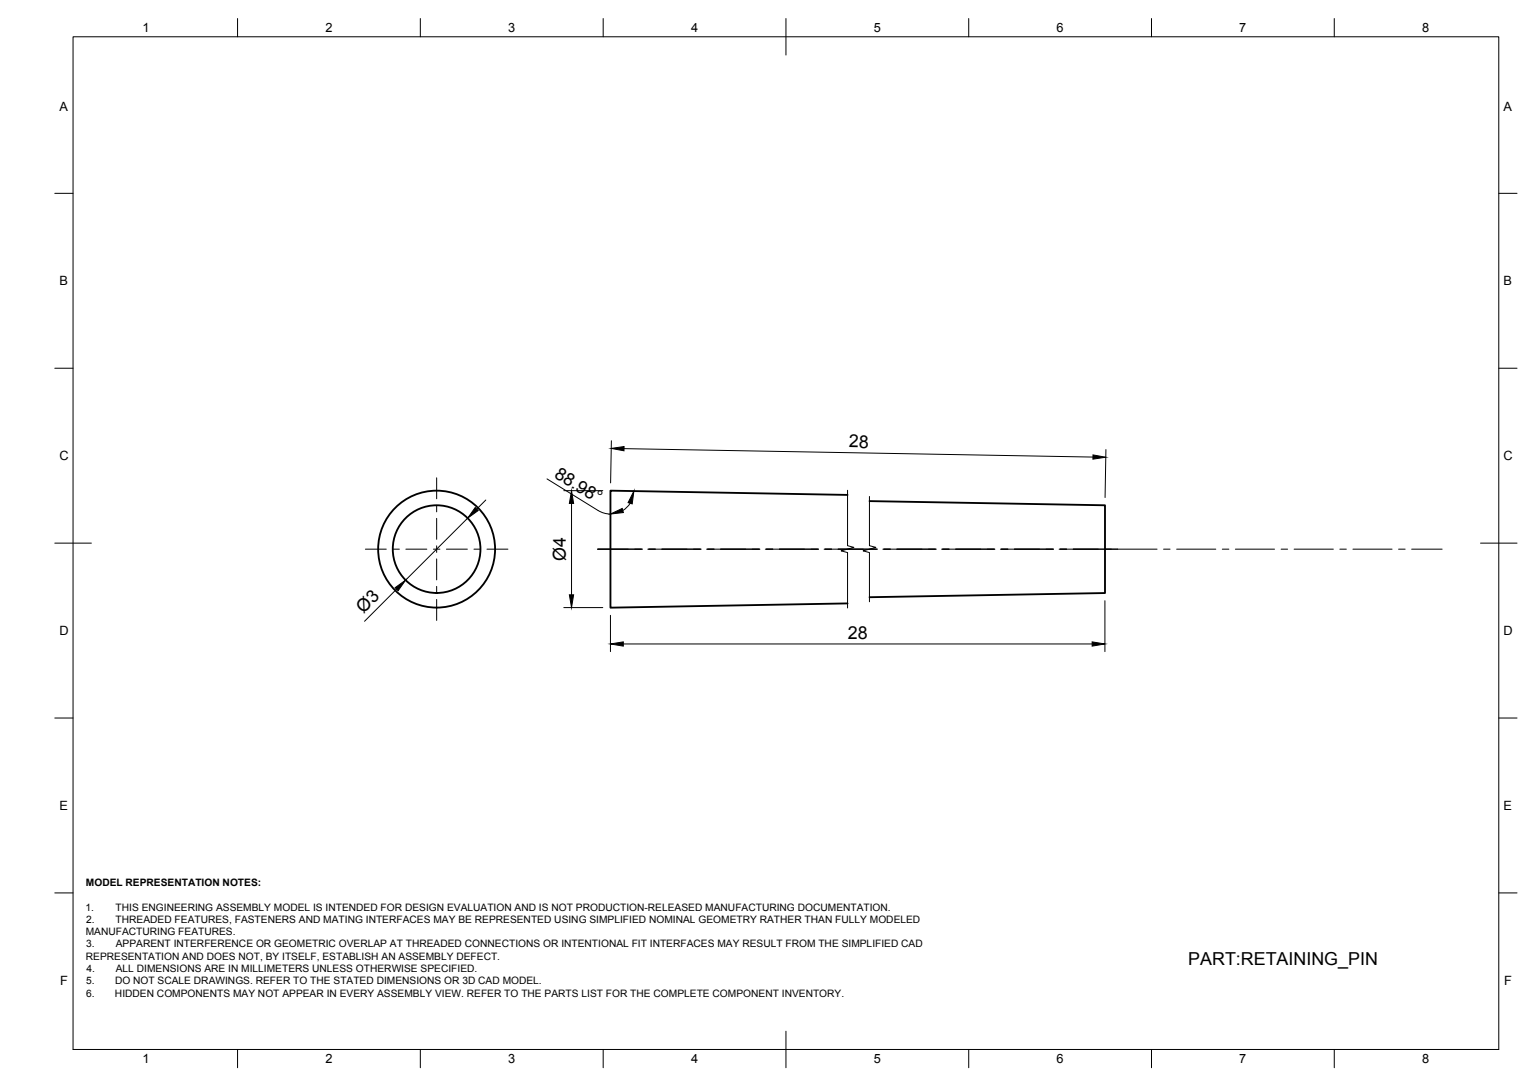
ISO-10303-21;
HEADER;
/* Generated by software containing ST-Developer
 * from STEP Tools, Inc. (www.steptools.com) 
 */

FILE_DESCRIPTION(
/* description */ (''),
/* implementation_level */ '2;1');

FILE_NAME(
/* name */ 'RETAINING_PIN.step',
/* time_stamp */ '2026-10-04T02:10:06-07:00',
/* author */ (''),
/* organization */ (''),
/* preprocessor_version */ 'ST-DEVELOPER v20.2',
/* originating_system */ 'Autodesk Translation Framework v15.15.0.0',
/* authorisation */ '');

FILE_SCHEMA (('AUTOMOTIVE_DESIGN { 1 0 10303 214 3 1 1 }'));
ENDSEC;

DATA;
#10=MECHANICAL_DESIGN_GEOMETRIC_PRESENTATION_REPRESENTATION('',(#145),#9668);
#123=SHAPE_REPRESENTATION_RELATIONSHIP('SRR','None',#9716,#134);
#134=ADVANCED_BREP_SHAPE_REPRESENTATION('',(#156),#9661);
#145=STYLED_ITEM('',(#9775),#156);
#156=MANIFOLD_SOLID_BREP('Body1',#3885);
#172=CONICAL_SURFACE('',#4235,1.5,0.0178552451395525);
#313=PLANE('',#4238);
#314=PLANE('',#4239);
#472=LINE('',#6770,#663);
#663=VECTOR('',#5016,1.5);
#911=FACE_OUTER_BOUND('',#1180,.T.);
#912=FACE_OUTER_BOUND('',#1181,.T.);
#913=FACE_OUTER_BOUND('',#1182,.T.);
#1180=EDGE_LOOP('',(#3047,#3048,#3049,#3050));
#1181=EDGE_LOOP('',(#3051));
#1182=EDGE_LOOP('',(#3052));
#1541=CIRCLE('',#4236,2.);
#1542=CIRCLE('',#4237,1.5);
#1807=VERTEX_POINT('',#6767);
#1808=VERTEX_POINT('',#6769);
#2247=EDGE_CURVE('',#1807,#1807,#1541,.T.);
#2248=EDGE_CURVE('',#1807,#1808,#472,.T.);
#2249=EDGE_CURVE('',#1808,#1808,#1542,.T.);
#3047=ORIENTED_EDGE('',*,*,#2247,.T.);
#3048=ORIENTED_EDGE('',*,*,#2248,.T.);
#3049=ORIENTED_EDGE('',*,*,#2249,.F.);
#3050=ORIENTED_EDGE('',*,*,#2248,.F.);
#3051=ORIENTED_EDGE('',*,*,#2247,.F.);
#3052=ORIENTED_EDGE('',*,*,#2249,.T.);
#3759=ADVANCED_FACE('',(#911),#172,.T.);
#3760=ADVANCED_FACE('',(#912),#313,.T.);
#3761=ADVANCED_FACE('',(#913),#314,.T.);
#3885=CLOSED_SHELL('',(#3759,#3760,#3761));
#4234=AXIS2_PLACEMENT_3D('',#6765,#5010,#5011);
#4235=AXIS2_PLACEMENT_3D('',#6766,#5012,#5013);
#4236=AXIS2_PLACEMENT_3D('',#6768,#5014,#5015);
#4237=AXIS2_PLACEMENT_3D('',#6771,#5017,#5018);
#4238=AXIS2_PLACEMENT_3D('',#6772,#5019,#5020);
#4239=AXIS2_PLACEMENT_3D('',#6773,#5021,#5022);
#5010=DIRECTION('axis',(0.,0.,1.));
#5011=DIRECTION('refdir',(1.,0.,0.));
#5012=DIRECTION('center_axis',(1.,0.,0.));
#5013=DIRECTION('ref_axis',(0.,0.,-1.));
#5014=DIRECTION('center_axis',(-1.,0.,0.));
#5015=DIRECTION('ref_axis',(0.,0.,1.));
#5016=DIRECTION('',(-0.999840599345445,2.18652069579637E-18,-0.0178542964168829));
#5017=DIRECTION('center_axis',(-1.,0.,0.));
#5018=DIRECTION('ref_axis',(0.,0.,1.));
#5019=DIRECTION('center_axis',(1.,0.,0.));
#5020=DIRECTION('ref_axis',(0.,0.,-1.));
#5021=DIRECTION('center_axis',(-1.,0.,0.));
#5022=DIRECTION('ref_axis',(0.,0.,1.));
#6765=CARTESIAN_POINT('',(0.,0.,0.));
#6766=CARTESIAN_POINT('Origin',(0.,0.,0.));
#6767=CARTESIAN_POINT('',(28.,0.,2.));
#6768=CARTESIAN_POINT('Origin',(28.,0.,0.));
#6769=CARTESIAN_POINT('',(0.,0.,1.5));
#6770=CARTESIAN_POINT('',(0.,-1.83697019872103E-16,1.5));
#6771=CARTESIAN_POINT('Origin',(0.,0.,0.));
#6772=CARTESIAN_POINT('Origin',(27.9999999999979,-2.,0.));
#6773=CARTESIAN_POINT('Origin',(-1.14810637420064E-16,0.,0.));
#9648=UNCERTAINTY_MEASURE_WITH_UNIT(LENGTH_MEASURE(0.01),#9669,
'DISTANCE_ACCURACY_VALUE',
'Maximum model space distance between geometric entities at asserted c
onnectivities');
#9655=UNCERTAINTY_MEASURE_WITH_UNIT(LENGTH_MEASURE(0.01),#9669,
'DISTANCE_ACCURACY_VALUE',
'Maximum model space distance between geometric entities at asserted c
onnectivities');
#9661=(
GEOMETRIC_REPRESENTATION_CONTEXT(3)
GLOBAL_UNCERTAINTY_ASSIGNED_CONTEXT((#9648))
GLOBAL_UNIT_ASSIGNED_CONTEXT((#9669,#9671,#9672))
REPRESENTATION_CONTEXT('','3D')
);
#9668=(
GEOMETRIC_REPRESENTATION_CONTEXT(3)
GLOBAL_UNCERTAINTY_ASSIGNED_CONTEXT((#9655))
GLOBAL_UNIT_ASSIGNED_CONTEXT((#9669,#9671,#9672))
REPRESENTATION_CONTEXT('','3D')
);
#9669=(
LENGTH_UNIT()
NAMED_UNIT(*)
SI_UNIT(.MILLI.,.METRE.)
);
#9671=(
NAMED_UNIT(*)
PLANE_ANGLE_UNIT()
SI_UNIT($,.RADIAN.)
);
#9672=(
NAMED_UNIT(*)
SI_UNIT($,.STERADIAN.)
SOLID_ANGLE_UNIT()
);
#9678=SHAPE_DEFINITION_REPRESENTATION(#9690,#9716);
#9690=PRODUCT_DEFINITION_SHAPE('',$,#9729);
#9716=SHAPE_REPRESENTATION('',(#4234),#9661);
#9723=PRODUCT_DEFINITION_CONTEXT('part definition',#9761,'design');
#9729=PRODUCT_DEFINITION('2026-10-04-08-13-48-884','RETAINING_PIN',#9741,
#9723);
#9741=PRODUCT_DEFINITION_FORMATION('',$,#9768);
#9761=APPLICATION_CONTEXT(
'Core Data for Automotive Mechanical Design Process');
#9762=PRODUCT_CONTEXT('part definition',#9761,'mechanical');
#9768=PRODUCT('2026-10-04-08-13-48-884','RETAINING_PIN','PART',(#9762));
#9775=PRESENTATION_STYLE_ASSIGNMENT((#9776));
#9776=SURFACE_STYLE_USAGE(.BOTH.,#9777);
#9777=SURFACE_SIDE_STYLE('',(#9778));
#9778=SURFACE_STYLE_FILL_AREA(#9779);
#9779=FILL_AREA_STYLE('Steel - Satin',(#9780));
#9780=FILL_AREA_STYLE_COLOUR('Steel - Satin',#9781);
#9781=COLOUR_RGB('Steel - Satin', 0.09019608, 0.27058824, 0.51372549);
ENDSEC;
END-ISO-10303-21;
